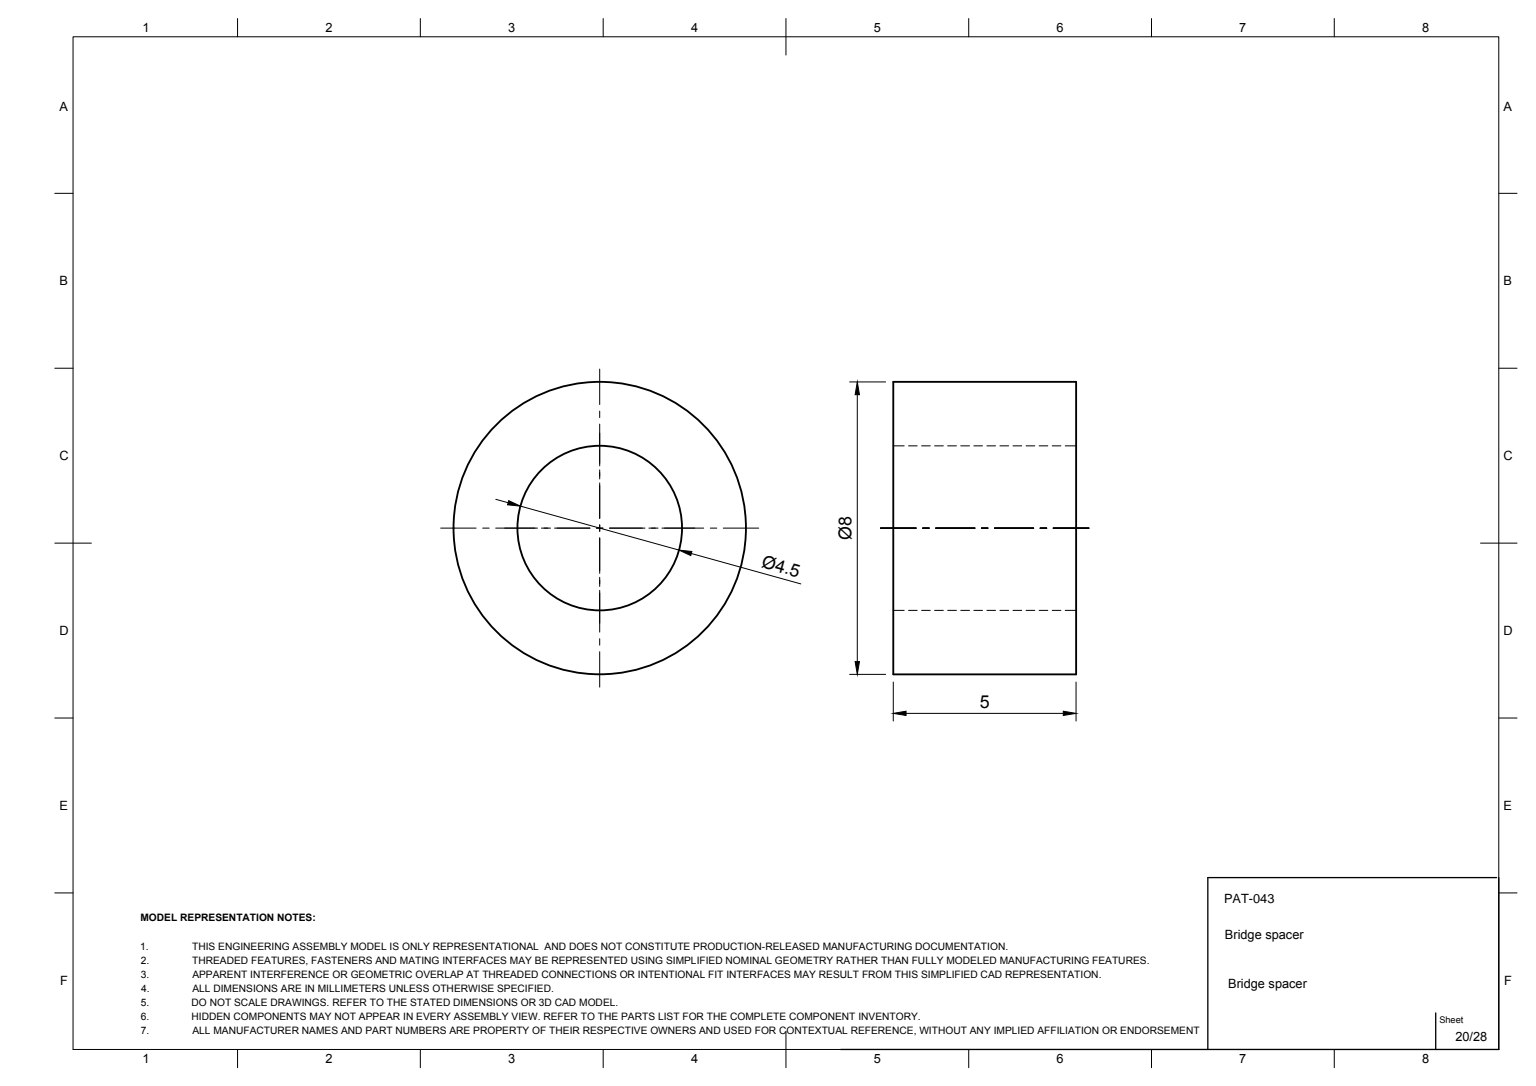
ISO-10303-21;
HEADER;
/* Generated by software containing ST-Developer
 * from STEP Tools, Inc. (www.steptools.com) 
 */

FILE_DESCRIPTION(
/* description */ ('Four-valve pipe header'),
/* implementation_level */ '2;1');

FILE_NAME(
/* name */ 'Bridge spacer.step',
/* time_stamp */ '2026-10-29T16:56:19-07:00',
/* author */ (''),
/* organization */ (''),
/* preprocessor_version */ 'ST-DEVELOPER v20.2',
/* originating_system */ 'Autodesk Translation Framework v15.17.0.0',
/* authorisation */ '');

FILE_SCHEMA (('AUTOMOTIVE_DESIGN { 1 0 10303 214 3 1 1 }'));
ENDSEC;

DATA;
#10=MECHANICAL_DESIGN_GEOMETRIC_PRESENTATION_REPRESENTATION('',(#350),#10119);
#298=SHAPE_REPRESENTATION_RELATIONSHIP('SRR','None',#10260,#324);
#324=ADVANCED_BREP_SHAPE_REPRESENTATION('',(#375),#10109);
#350=STYLED_ITEM('',(#10463),#375);
#375=MANIFOLD_SOLID_BREP('Body1',#5597);
#523=FACE_BOUND('',#1422,.T.);
#524=FACE_BOUND('',#1424,.T.);
#678=PLANE('',#6376);
#679=PLANE('',#6377);
#990=FACE_OUTER_BOUND('',#1419,.T.);
#991=FACE_OUTER_BOUND('',#1420,.T.);
#992=FACE_OUTER_BOUND('',#1421,.T.);
#993=FACE_OUTER_BOUND('',#1423,.T.);
#1419=EDGE_LOOP('',(#4797,#4798,#4799,#4800));
#1420=EDGE_LOOP('',(#4801,#4802,#4803,#4804));
#1421=EDGE_LOOP('',(#4805));
#1422=EDGE_LOOP('',(#4806));
#1423=EDGE_LOOP('',(#4807));
#1424=EDGE_LOOP('',(#4808));
#1807=LINE('',#9619,#2225);
#1808=LINE('',#9625,#2226);
#2225=VECTOR('',#7810,0.225);
#2226=VECTOR('',#7817,0.4);
#2535=CIRCLE('',#6371,0.225);
#2536=CIRCLE('',#6372,0.225);
#2537=CIRCLE('',#6374,0.4);
#2538=CIRCLE('',#6375,0.4);
#2924=VERTEX_POINT('',#9616);
#2925=VERTEX_POINT('',#9618);
#2926=VERTEX_POINT('',#9622);
#2927=VERTEX_POINT('',#9624);
#3565=EDGE_CURVE('',#2924,#2924,#2535,.T.);
#3566=EDGE_CURVE('',#2924,#2925,#1807,.T.);
#3567=EDGE_CURVE('',#2925,#2925,#2536,.T.);
#3568=EDGE_CURVE('',#2926,#2926,#2537,.T.);
#3569=EDGE_CURVE('',#2926,#2927,#1808,.T.);
#3570=EDGE_CURVE('',#2927,#2927,#2538,.T.);
#4797=ORIENTED_EDGE('',*,*,#3565,.F.);
#4798=ORIENTED_EDGE('',*,*,#3566,.T.);
#4799=ORIENTED_EDGE('',*,*,#3567,.T.);
#4800=ORIENTED_EDGE('',*,*,#3566,.F.);
#4801=ORIENTED_EDGE('',*,*,#3568,.F.);
#4802=ORIENTED_EDGE('',*,*,#3569,.T.);
#4803=ORIENTED_EDGE('',*,*,#3570,.T.);
#4804=ORIENTED_EDGE('',*,*,#3569,.F.);
#4805=ORIENTED_EDGE('',*,*,#3568,.T.);
#4806=ORIENTED_EDGE('',*,*,#3565,.T.);
#4807=ORIENTED_EDGE('',*,*,#3570,.F.);
#4808=ORIENTED_EDGE('',*,*,#3567,.F.);
#5235=CYLINDRICAL_SURFACE('',#6370,0.225);
#5236=CYLINDRICAL_SURFACE('',#6373,0.4);
#5490=ADVANCED_FACE('',(#990),#5235,.F.);
#5491=ADVANCED_FACE('',(#991),#5236,.T.);
#5492=ADVANCED_FACE('',(#992,#523),#678,.T.);
#5493=ADVANCED_FACE('',(#993,#524),#679,.F.);
#5597=CLOSED_SHELL('',(#5490,#5491,#5492,#5493));
#6369=AXIS2_PLACEMENT_3D('',#9614,#7804,#7805);
#6370=AXIS2_PLACEMENT_3D('',#9615,#7806,#7807);
#6371=AXIS2_PLACEMENT_3D('',#9617,#7808,#7809);
#6372=AXIS2_PLACEMENT_3D('',#9620,#7811,#7812);
#6373=AXIS2_PLACEMENT_3D('',#9621,#7813,#7814);
#6374=AXIS2_PLACEMENT_3D('',#9623,#7815,#7816);
#6375=AXIS2_PLACEMENT_3D('',#9626,#7818,#7819);
#6376=AXIS2_PLACEMENT_3D('',#9627,#7820,#7821);
#6377=AXIS2_PLACEMENT_3D('',#9628,#7822,#7823);
#7804=DIRECTION('axis',(0.,0.,1.));
#7805=DIRECTION('refdir',(1.,0.,0.));
#7806=DIRECTION('center_axis',(0.,0.,1.));
#7807=DIRECTION('ref_axis',(1.,0.,0.));
#7808=DIRECTION('center_axis',(0.,0.,-1.));
#7809=DIRECTION('ref_axis',(1.,0.,0.));
#7810=DIRECTION('',(0.,0.,-1.));
#7811=DIRECTION('center_axis',(0.,0.,-1.));
#7812=DIRECTION('ref_axis',(1.,0.,0.));
#7813=DIRECTION('center_axis',(0.,0.,1.));
#7814=DIRECTION('ref_axis',(1.,0.,0.));
#7815=DIRECTION('center_axis',(0.,0.,1.));
#7816=DIRECTION('ref_axis',(1.,0.,0.));
#7817=DIRECTION('',(0.,0.,-1.));
#7818=DIRECTION('center_axis',(0.,0.,1.));
#7819=DIRECTION('ref_axis',(1.,0.,0.));
#7820=DIRECTION('center_axis',(0.,0.,1.));
#7821=DIRECTION('ref_axis',(1.,0.,0.));
#7822=DIRECTION('center_axis',(0.,0.,1.));
#7823=DIRECTION('ref_axis',(1.,0.,0.));
#9614=CARTESIAN_POINT('',(0.,0.,0.));
#9615=CARTESIAN_POINT('Origin',(-1.3,-1.,7.5));
#9616=CARTESIAN_POINT('',(-1.525,-1.,8.));
#9617=CARTESIAN_POINT('Origin',(-1.3,-1.,8.));
#9618=CARTESIAN_POINT('',(-1.525,-1.,7.5));
#9619=CARTESIAN_POINT('',(-1.525,-1.,7.5));
#9620=CARTESIAN_POINT('Origin',(-1.3,-1.,7.5));
#9621=CARTESIAN_POINT('Origin',(-1.3,-1.,7.5));
#9622=CARTESIAN_POINT('',(-1.7,-1.,8.));
#9623=CARTESIAN_POINT('Origin',(-1.3,-1.,8.));
#9624=CARTESIAN_POINT('',(-1.7,-1.,7.5));
#9625=CARTESIAN_POINT('',(-1.7,-1.,7.5));
#9626=CARTESIAN_POINT('Origin',(-1.3,-1.,7.5));
#9627=CARTESIAN_POINT('Origin',(-1.3,-1.,8.));
#9628=CARTESIAN_POINT('Origin',(-1.3,-1.,7.5));
#10078=UNCERTAINTY_MEASURE_WITH_UNIT(LENGTH_MEASURE(0.001),#10120,
'DISTANCE_ACCURACY_VALUE',
'Maximum model space distance between geometric entities at asserted c
onnectivities');
#10088=UNCERTAINTY_MEASURE_WITH_UNIT(LENGTH_MEASURE(0.001),#10120,
'DISTANCE_ACCURACY_VALUE',
'Maximum model space distance between geometric entities at asserted c
onnectivities');
#10109=(
GEOMETRIC_REPRESENTATION_CONTEXT(3)
GLOBAL_UNCERTAINTY_ASSIGNED_CONTEXT((#10078))
GLOBAL_UNIT_ASSIGNED_CONTEXT((#10120,#10122,#10123))
REPRESENTATION_CONTEXT('','3D')
);
#10119=(
GEOMETRIC_REPRESENTATION_CONTEXT(3)
GLOBAL_UNCERTAINTY_ASSIGNED_CONTEXT((#10088))
GLOBAL_UNIT_ASSIGNED_CONTEXT((#10120,#10122,#10123))
REPRESENTATION_CONTEXT('','3D')
);
#10120=(
LENGTH_UNIT()
NAMED_UNIT(*)
SI_UNIT(.CENTI.,.METRE.)
);
#10122=(
NAMED_UNIT(*)
PLANE_ANGLE_UNIT()
SI_UNIT($,.RADIAN.)
);
#10123=(
NAMED_UNIT(*)
SI_UNIT($,.STERADIAN.)
SOLID_ANGLE_UNIT()
);
#10144=SHAPE_DEFINITION_REPRESENTATION(#10174,#10260);
#10174=PRODUCT_DEFINITION_SHAPE('',$,#10291);
#10260=SHAPE_REPRESENTATION('',(#6369),#10109);
#10270=PRODUCT_DEFINITION_CONTEXT('part definition',#10362,'design');
#10291=PRODUCT_DEFINITION('Bridge spacer','Bridge spacer',#10321,#10270);
#10321=PRODUCT_DEFINITION_FORMATION('',$,#10384);
#10362=APPLICATION_CONTEXT(
'Core Data for Automotive Mechanical Design Process');
#10363=PRODUCT_CONTEXT('part definition',#10362,'mechanical');
#10384=PRODUCT('Bridge spacer','Bridge spacer','Bridge spacer',(#10363));
#10457=COLOUR_RGB('Sky Blue',0.24,0.69,0.87);
#10458=FILL_AREA_STYLE_COLOUR('',#10457);
#10459=FILL_AREA_STYLE('',(#10458));
#10460=SURFACE_STYLE_FILL_AREA(#10459);
#10461=SURFACE_SIDE_STYLE('',(#10460));
#10462=SURFACE_STYLE_USAGE(.BOTH.,#10461);
#10463=PRESENTATION_STYLE_ASSIGNMENT((#10462));
ENDSEC;
END-ISO-10303-21;
